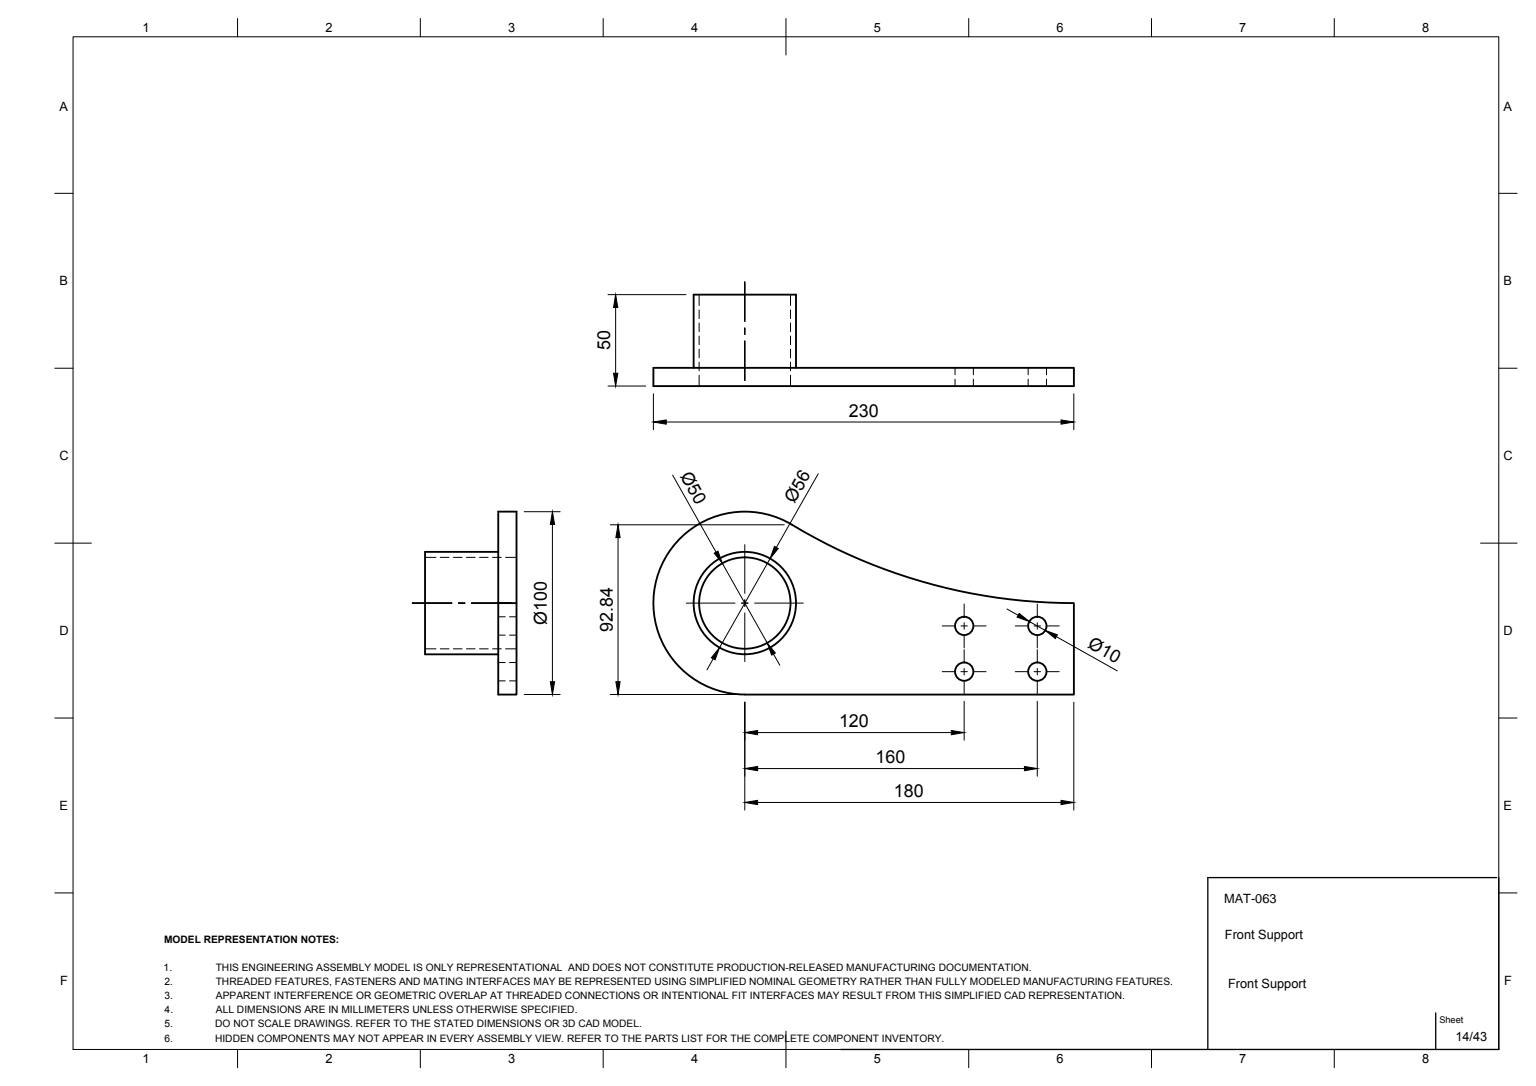
ISO-10303-21;
HEADER;
/* Generated by software containing ST-Developer
 * from STEP Tools, Inc. (www.steptools.com) 
 */

FILE_DESCRIPTION(
/* description */ (''),
/* implementation_level */ '2;1');

FILE_NAME(
/* name */ 'Front Support.step',
/* time_stamp */ '2026-10-24T09:43:01-07:00',
/* author */ (''),
/* organization */ (''),
/* preprocessor_version */ 'ST-DEVELOPER v20.2',
/* originating_system */ 'Autodesk Translation Framework v15.15.0.0',
/* authorisation */ '');

FILE_SCHEMA (('AUTOMOTIVE_DESIGN { 1 0 10303 214 3 1 1 }'));
ENDSEC;

DATA;
#10=MECHANICAL_DESIGN_GEOMETRIC_PRESENTATION_REPRESENTATION('',(#302),#11112);
#236=SHAPE_REPRESENTATION_RELATIONSHIP('SRR','None',#11262,#269);
#269=ADVANCED_BREP_SHAPE_REPRESENTATION('',(#335),#11107);
#302=STYLED_ITEM('',(#11426),#335);
#335=MANIFOLD_SOLID_BREP('Front Support',#6039);
#481=FACE_BOUND('',#1521,.T.);
#482=FACE_BOUND('',#1523,.T.);
#483=FACE_BOUND('',#1524,.T.);
#484=FACE_BOUND('',#1525,.T.);
#485=FACE_BOUND('',#1526,.T.);
#486=FACE_BOUND('',#1527,.T.);
#487=FACE_BOUND('',#1538,.T.);
#488=FACE_BOUND('',#1539,.T.);
#489=FACE_BOUND('',#1540,.T.);
#490=FACE_BOUND('',#1541,.T.);
#491=FACE_BOUND('',#1542,.T.);
#654=PLANE('',#7190);
#655=PLANE('',#7192);
#656=PLANE('',#7209);
#657=PLANE('',#7214);
#658=PLANE('',#7215);
#1013=FACE_OUTER_BOUND('',#1519,.T.);
#1014=FACE_OUTER_BOUND('',#1520,.T.);
#1015=FACE_OUTER_BOUND('',#1522,.T.);
#1016=FACE_OUTER_BOUND('',#1528,.T.);
#1017=FACE_OUTER_BOUND('',#1529,.T.);
#1018=FACE_OUTER_BOUND('',#1530,.T.);
#1019=FACE_OUTER_BOUND('',#1531,.T.);
#1020=FACE_OUTER_BOUND('',#1532,.T.);
#1021=FACE_OUTER_BOUND('',#1533,.T.);
#1022=FACE_OUTER_BOUND('',#1534,.T.);
#1023=FACE_OUTER_BOUND('',#1535,.T.);
#1024=FACE_OUTER_BOUND('',#1536,.T.);
#1025=FACE_OUTER_BOUND('',#1537,.T.);
#1519=EDGE_LOOP('',(#5409,#5410,#5411,#5412));
#1520=EDGE_LOOP('',(#5413));
#1521=EDGE_LOOP('',(#5414));
#1522=EDGE_LOOP('',(#5415,#5416,#5417,#5418));
#1523=EDGE_LOOP('',(#5419));
#1524=EDGE_LOOP('',(#5420));
#1525=EDGE_LOOP('',(#5421));
#1526=EDGE_LOOP('',(#5422));
#1527=EDGE_LOOP('',(#5423));
#1528=EDGE_LOOP('',(#5424,#5425,#5426,#5427));
#1529=EDGE_LOOP('',(#5428,#5429,#5430,#5431));
#1530=EDGE_LOOP('',(#5432,#5433,#5434,#5435));
#1531=EDGE_LOOP('',(#5436,#5437,#5438,#5439));
#1532=EDGE_LOOP('',(#5440,#5441,#5442,#5443));
#1533=EDGE_LOOP('',(#5444,#5445,#5446,#5447));
#1534=EDGE_LOOP('',(#5448,#5449,#5450,#5451));
#1535=EDGE_LOOP('',(#5452,#5453,#5454,#5455));
#1536=EDGE_LOOP('',(#5456,#5457,#5458,#5459));
#1537=EDGE_LOOP('',(#5460,#5461,#5462,#5463));
#1538=EDGE_LOOP('',(#5464));
#1539=EDGE_LOOP('',(#5465));
#1540=EDGE_LOOP('',(#5466));
#1541=EDGE_LOOP('',(#5467));
#1542=EDGE_LOOP('',(#5468));
#1898=LINE('',#10917,#2257);
#1899=LINE('',#10925,#2258);
#1900=LINE('',#10927,#2259);
#1901=LINE('',#10942,#2260);
#1902=LINE('',#10946,#2261);
#1903=LINE('',#10950,#2262);
#1904=LINE('',#10954,#2263);
#1905=LINE('',#10958,#2264);
#1906=LINE('',#10961,#2265);
#1907=LINE('',#10963,#2266);
#1908=LINE('',#10964,#2267);
#1909=LINE('',#10968,#2268);
#1910=LINE('',#10971,#2269);
#1911=LINE('',#10974,#2270);
#2257=VECTOR('',#9164,0.028);
#2258=VECTOR('',#9173,0.01);
#2259=VECTOR('',#9174,0.01);
#2260=VECTOR('',#9191,0.025);
#2261=VECTOR('',#9196,0.0049999999999998);
#2262=VECTOR('',#9201,0.005);
#2263=VECTOR('',#9206,0.0049999999999998);
#2264=VECTOR('',#9211,0.005);
#2265=VECTOR('',#9214,0.01);
#2266=VECTOR('',#9215,0.01);
#2267=VECTOR('',#9216,0.01);
#2268=VECTOR('',#9221,0.01);
#2269=VECTOR('',#9224,0.01);
#2270=VECTOR('',#9229,0.01);
#2656=CIRCLE('',#7188,0.028);
#2657=CIRCLE('',#7189,0.028);
#2658=CIRCLE('',#7191,0.025);
#2659=CIRCLE('',#7193,0.299);
#2660=CIRCLE('',#7194,0.05);
#2661=CIRCLE('',#7195,0.005);
#2662=CIRCLE('',#7196,0.0049999999999998);
#2663=CIRCLE('',#7197,0.005);
#2664=CIRCLE('',#7198,0.0049999999999998);
#2665=CIRCLE('',#7200,0.025);
#2666=CIRCLE('',#7202,0.0049999999999998);
#2667=CIRCLE('',#7204,0.005);
#2668=CIRCLE('',#7206,0.0049999999999998);
#2669=CIRCLE('',#7208,0.005);
#2670=CIRCLE('',#7211,0.299);
#2671=CIRCLE('',#7213,0.05);
#3150=VERTEX_POINT('',#10914);
#3151=VERTEX_POINT('',#10916);
#3152=VERTEX_POINT('',#10920);
#3153=VERTEX_POINT('',#10923);
#3154=VERTEX_POINT('',#10924);
#3155=VERTEX_POINT('',#10926);
#3156=VERTEX_POINT('',#10928);
#3157=VERTEX_POINT('',#10931);
#3158=VERTEX_POINT('',#10933);
#3159=VERTEX_POINT('',#10935);
#3160=VERTEX_POINT('',#10937);
#3161=VERTEX_POINT('',#10940);
#3162=VERTEX_POINT('',#10944);
#3163=VERTEX_POINT('',#10948);
#3164=VERTEX_POINT('',#10952);
#3165=VERTEX_POINT('',#10956);
#3166=VERTEX_POINT('',#10960);
#3167=VERTEX_POINT('',#10962);
#3168=VERTEX_POINT('',#10966);
#3169=VERTEX_POINT('',#10970);
#3908=EDGE_CURVE('',#3150,#3150,#2656,.F.);
#3909=EDGE_CURVE('',#3150,#3151,#1898,.T.);
#3910=EDGE_CURVE('',#3151,#3151,#2657,.T.);
#3911=EDGE_CURVE('',#3152,#3152,#2658,.F.);
#3912=EDGE_CURVE('',#3153,#3154,#1899,.T.);
#3913=EDGE_CURVE('',#3155,#3153,#1900,.T.);
#3914=EDGE_CURVE('',#3156,#3155,#2659,.T.);
#3915=EDGE_CURVE('',#3154,#3156,#2660,.F.);
#3916=EDGE_CURVE('',#3157,#3157,#2661,.T.);
#3917=EDGE_CURVE('',#3158,#3158,#2662,.T.);
#3918=EDGE_CURVE('',#3159,#3159,#2663,.T.);
#3919=EDGE_CURVE('',#3160,#3160,#2664,.T.);
#3920=EDGE_CURVE('',#3161,#3161,#2665,.T.);
#3921=EDGE_CURVE('',#3161,#3152,#1901,.T.);
#3922=EDGE_CURVE('',#3162,#3162,#2666,.T.);
#3923=EDGE_CURVE('',#3162,#3160,#1902,.T.);
#3924=EDGE_CURVE('',#3163,#3163,#2667,.T.);
#3925=EDGE_CURVE('',#3163,#3159,#1903,.T.);
#3926=EDGE_CURVE('',#3164,#3164,#2668,.T.);
#3927=EDGE_CURVE('',#3164,#3158,#1904,.T.);
#3928=EDGE_CURVE('',#3165,#3165,#2669,.T.);
#3929=EDGE_CURVE('',#3165,#3157,#1905,.T.);
#3930=EDGE_CURVE('',#3155,#3166,#1906,.T.);
#3931=EDGE_CURVE('',#3167,#3153,#1907,.T.);
#3932=EDGE_CURVE('',#3166,#3167,#1908,.T.);
#3933=EDGE_CURVE('',#3168,#3166,#2670,.T.);
#3934=EDGE_CURVE('',#3156,#3168,#1909,.F.);
#3935=EDGE_CURVE('',#3169,#3154,#1910,.F.);
#3936=EDGE_CURVE('',#3168,#3169,#2671,.T.);
#3937=EDGE_CURVE('',#3169,#3167,#1911,.T.);
#5409=ORIENTED_EDGE('',*,*,#3908,.T.);
#5410=ORIENTED_EDGE('',*,*,#3909,.T.);
#5411=ORIENTED_EDGE('',*,*,#3910,.T.);
#5412=ORIENTED_EDGE('',*,*,#3909,.F.);
#5413=ORIENTED_EDGE('',*,*,#3910,.F.);
#5414=ORIENTED_EDGE('',*,*,#3911,.T.);
#5415=ORIENTED_EDGE('',*,*,#3912,.F.);
#5416=ORIENTED_EDGE('',*,*,#3913,.F.);
#5417=ORIENTED_EDGE('',*,*,#3914,.F.);
#5418=ORIENTED_EDGE('',*,*,#3915,.F.);
#5419=ORIENTED_EDGE('',*,*,#3916,.F.);
#5420=ORIENTED_EDGE('',*,*,#3917,.F.);
#5421=ORIENTED_EDGE('',*,*,#3918,.F.);
#5422=ORIENTED_EDGE('',*,*,#3919,.F.);
#5423=ORIENTED_EDGE('',*,*,#3908,.F.);
#5424=ORIENTED_EDGE('',*,*,#3920,.F.);
#5425=ORIENTED_EDGE('',*,*,#3921,.T.);
#5426=ORIENTED_EDGE('',*,*,#3911,.F.);
#5427=ORIENTED_EDGE('',*,*,#3921,.F.);
#5428=ORIENTED_EDGE('',*,*,#3922,.F.);
#5429=ORIENTED_EDGE('',*,*,#3923,.T.);
#5430=ORIENTED_EDGE('',*,*,#3919,.T.);
#5431=ORIENTED_EDGE('',*,*,#3923,.F.);
#5432=ORIENTED_EDGE('',*,*,#3924,.F.);
#5433=ORIENTED_EDGE('',*,*,#3925,.T.);
#5434=ORIENTED_EDGE('',*,*,#3918,.T.);
#5435=ORIENTED_EDGE('',*,*,#3925,.F.);
#5436=ORIENTED_EDGE('',*,*,#3926,.F.);
#5437=ORIENTED_EDGE('',*,*,#3927,.T.);
#5438=ORIENTED_EDGE('',*,*,#3917,.T.);
#5439=ORIENTED_EDGE('',*,*,#3927,.F.);
#5440=ORIENTED_EDGE('',*,*,#3928,.F.);
#5441=ORIENTED_EDGE('',*,*,#3929,.T.);
#5442=ORIENTED_EDGE('',*,*,#3916,.T.);
#5443=ORIENTED_EDGE('',*,*,#3929,.F.);
#5444=ORIENTED_EDGE('',*,*,#3930,.F.);
#5445=ORIENTED_EDGE('',*,*,#3913,.T.);
#5446=ORIENTED_EDGE('',*,*,#3931,.F.);
#5447=ORIENTED_EDGE('',*,*,#3932,.F.);
#5448=ORIENTED_EDGE('',*,*,#3914,.T.);
#5449=ORIENTED_EDGE('',*,*,#3930,.T.);
#5450=ORIENTED_EDGE('',*,*,#3933,.F.);
#5451=ORIENTED_EDGE('',*,*,#3934,.F.);
#5452=ORIENTED_EDGE('',*,*,#3935,.T.);
#5453=ORIENTED_EDGE('',*,*,#3915,.T.);
#5454=ORIENTED_EDGE('',*,*,#3934,.T.);
#5455=ORIENTED_EDGE('',*,*,#3936,.T.);
#5456=ORIENTED_EDGE('',*,*,#3912,.T.);
#5457=ORIENTED_EDGE('',*,*,#3935,.F.);
#5458=ORIENTED_EDGE('',*,*,#3937,.T.);
#5459=ORIENTED_EDGE('',*,*,#3931,.T.);
#5460=ORIENTED_EDGE('',*,*,#3932,.T.);
#5461=ORIENTED_EDGE('',*,*,#3937,.F.);
#5462=ORIENTED_EDGE('',*,*,#3936,.F.);
#5463=ORIENTED_EDGE('',*,*,#3933,.T.);
#5464=ORIENTED_EDGE('',*,*,#3928,.T.);
#5465=ORIENTED_EDGE('',*,*,#3922,.T.);
#5466=ORIENTED_EDGE('',*,*,#3924,.T.);
#5467=ORIENTED_EDGE('',*,*,#3926,.T.);
#5468=ORIENTED_EDGE('',*,*,#3920,.T.);
#5633=CYLINDRICAL_SURFACE('',#7187,0.028);
#5634=CYLINDRICAL_SURFACE('',#7199,0.025);
#5635=CYLINDRICAL_SURFACE('',#7201,0.0049999999999998);
#5636=CYLINDRICAL_SURFACE('',#7203,0.005);
#5637=CYLINDRICAL_SURFACE('',#7205,0.0049999999999998);
#5638=CYLINDRICAL_SURFACE('',#7207,0.005);
#5639=CYLINDRICAL_SURFACE('',#7210,0.299);
#5640=CYLINDRICAL_SURFACE('',#7212,0.05);
#5986=ADVANCED_FACE('',(#1013),#5633,.T.);
#5987=ADVANCED_FACE('',(#1014,#481),#654,.T.);
#5988=ADVANCED_FACE('',(#1015,#482,#483,#484,#485,#486),#655,.F.);
#5989=ADVANCED_FACE('',(#1016),#5634,.F.);
#5990=ADVANCED_FACE('',(#1017),#5635,.F.);
#5991=ADVANCED_FACE('',(#1018),#5636,.F.);
#5992=ADVANCED_FACE('',(#1019),#5637,.F.);
#5993=ADVANCED_FACE('',(#1020),#5638,.F.);
#5994=ADVANCED_FACE('',(#1021),#656,.F.);
#5995=ADVANCED_FACE('',(#1022),#5639,.F.);
#5996=ADVANCED_FACE('',(#1023),#5640,.T.);
#5997=ADVANCED_FACE('',(#1024),#657,.T.);
#5998=ADVANCED_FACE('',(#1025,#487,#488,#489,#490,#491),#658,.T.);
#6039=CLOSED_SHELL('',(#5986,#5987,#5988,#5989,#5990,#5991,#5992,#5993,
#5994,#5995,#5996,#5997,#5998));
#7186=AXIS2_PLACEMENT_3D('',#10912,#9158,#9159);
#7187=AXIS2_PLACEMENT_3D('',#10913,#9160,#9161);
#7188=AXIS2_PLACEMENT_3D('',#10915,#9162,#9163);
#7189=AXIS2_PLACEMENT_3D('',#10918,#9165,#9166);
#7190=AXIS2_PLACEMENT_3D('',#10919,#9167,#9168);
#7191=AXIS2_PLACEMENT_3D('',#10921,#9169,#9170);
#7192=AXIS2_PLACEMENT_3D('',#10922,#9171,#9172);
#7193=AXIS2_PLACEMENT_3D('',#10929,#9175,#9176);
#7194=AXIS2_PLACEMENT_3D('',#10930,#9177,#9178);
#7195=AXIS2_PLACEMENT_3D('',#10932,#9179,#9180);
#7196=AXIS2_PLACEMENT_3D('',#10934,#9181,#9182);
#7197=AXIS2_PLACEMENT_3D('',#10936,#9183,#9184);
#7198=AXIS2_PLACEMENT_3D('',#10938,#9185,#9186);
#7199=AXIS2_PLACEMENT_3D('',#10939,#9187,#9188);
#7200=AXIS2_PLACEMENT_3D('',#10941,#9189,#9190);
#7201=AXIS2_PLACEMENT_3D('',#10943,#9192,#9193);
#7202=AXIS2_PLACEMENT_3D('',#10945,#9194,#9195);
#7203=AXIS2_PLACEMENT_3D('',#10947,#9197,#9198);
#7204=AXIS2_PLACEMENT_3D('',#10949,#9199,#9200);
#7205=AXIS2_PLACEMENT_3D('',#10951,#9202,#9203);
#7206=AXIS2_PLACEMENT_3D('',#10953,#9204,#9205);
#7207=AXIS2_PLACEMENT_3D('',#10955,#9207,#9208);
#7208=AXIS2_PLACEMENT_3D('',#10957,#9209,#9210);
#7209=AXIS2_PLACEMENT_3D('',#10959,#9212,#9213);
#7210=AXIS2_PLACEMENT_3D('',#10965,#9217,#9218);
#7211=AXIS2_PLACEMENT_3D('',#10967,#9219,#9220);
#7212=AXIS2_PLACEMENT_3D('',#10969,#9222,#9223);
#7213=AXIS2_PLACEMENT_3D('',#10972,#9225,#9226);
#7214=AXIS2_PLACEMENT_3D('',#10973,#9227,#9228);
#7215=AXIS2_PLACEMENT_3D('',#10975,#9230,#9231);
#9158=DIRECTION('axis',(0.,0.,1.));
#9159=DIRECTION('refdir',(1.,0.,0.));
#9160=DIRECTION('center_axis',(-1.,0.,0.));
#9161=DIRECTION('ref_axis',(0.,0.,1.));
#9162=DIRECTION('center_axis',(-1.,0.,0.));
#9163=DIRECTION('ref_axis',(0.,0.,1.));
#9164=DIRECTION('',(1.,0.,0.));
#9165=DIRECTION('center_axis',(-1.,0.,0.));
#9166=DIRECTION('ref_axis',(0.,0.,1.));
#9167=DIRECTION('center_axis',(1.,-9.9268665898833E-16,1.01959257413342E-15));
#9168=DIRECTION('ref_axis',(1.01959257413342E-15,0.,-1.));
#9169=DIRECTION('center_axis',(1.,0.,0.));
#9170=DIRECTION('ref_axis',(0.,0.,-1.));
#9171=DIRECTION('center_axis',(-1.,0.,0.));
#9172=DIRECTION('ref_axis',(0.,0.,1.));
#9173=DIRECTION('',(0.,0.,1.));
#9174=DIRECTION('',(0.,-1.,1.98951966438983E-14));
#9175=DIRECTION('center_axis',(1.,0.,0.));
#9176=DIRECTION('ref_axis',(0.,0.,-1.));
#9177=DIRECTION('center_axis',(1.,0.,0.));
#9178=DIRECTION('ref_axis',(0.,0.,-1.));
#9179=DIRECTION('center_axis',(1.,0.,0.));
#9180=DIRECTION('ref_axis',(0.,0.,-1.));
#9181=DIRECTION('center_axis',(1.,0.,0.));
#9182=DIRECTION('ref_axis',(0.,0.,-1.));
#9183=DIRECTION('center_axis',(1.,0.,0.));
#9184=DIRECTION('ref_axis',(0.,0.,-1.));
#9185=DIRECTION('center_axis',(1.,0.,0.));
#9186=DIRECTION('ref_axis',(0.,0.,-1.));
#9187=DIRECTION('center_axis',(1.,0.,0.));
#9188=DIRECTION('ref_axis',(0.,0.,-1.));
#9189=DIRECTION('center_axis',(1.,0.,0.));
#9190=DIRECTION('ref_axis',(0.,0.,-1.));
#9191=DIRECTION('',(1.,0.,0.));
#9192=DIRECTION('center_axis',(1.,0.,0.));
#9193=DIRECTION('ref_axis',(0.,0.,-1.));
#9194=DIRECTION('center_axis',(1.,0.,0.));
#9195=DIRECTION('ref_axis',(0.,0.,-1.));
#9196=DIRECTION('',(1.,0.,0.));
#9197=DIRECTION('center_axis',(1.,0.,0.));
#9198=DIRECTION('ref_axis',(0.,0.,-1.));
#9199=DIRECTION('center_axis',(1.,0.,0.));
#9200=DIRECTION('ref_axis',(0.,0.,-1.));
#9201=DIRECTION('',(1.,0.,0.));
#9202=DIRECTION('center_axis',(1.,0.,0.));
#9203=DIRECTION('ref_axis',(0.,0.,-1.));
#9204=DIRECTION('center_axis',(1.,0.,0.));
#9205=DIRECTION('ref_axis',(0.,0.,-1.));
#9206=DIRECTION('',(1.,0.,0.));
#9207=DIRECTION('center_axis',(1.,0.,0.));
#9208=DIRECTION('ref_axis',(0.,0.,-1.));
#9209=DIRECTION('center_axis',(1.,0.,0.));
#9210=DIRECTION('ref_axis',(0.,0.,-1.));
#9211=DIRECTION('',(1.,0.,0.));
#9212=DIRECTION('center_axis',(2.20458572024499E-15,5.64627709665039E-16,
1.));
#9213=DIRECTION('ref_axis',(1.,5.1073991127734E-47,-2.20458572024499E-15));
#9214=DIRECTION('',(-1.,0.,0.));
#9215=DIRECTION('',(1.,0.,0.));
#9216=DIRECTION('',(0.,-1.,0.));
#9217=DIRECTION('center_axis',(1.,0.,0.));
#9218=DIRECTION('ref_axis',(0.,0.,-1.));
#9219=DIRECTION('center_axis',(1.,0.,0.));
#9220=DIRECTION('ref_axis',(0.,0.,-1.));
#9221=DIRECTION('',(1.,0.,0.));
#9222=DIRECTION('center_axis',(1.,0.,0.));
#9223=DIRECTION('ref_axis',(0.,0.267643864798619,0.963517909348684));
#9224=DIRECTION('',(-1.,0.,0.));
#9225=DIRECTION('center_axis',(1.,0.,0.));
#9226=DIRECTION('ref_axis',(0.,0.,-1.));
#9227=DIRECTION('center_axis',(3.68752646949032E-16,-1.,-1.69617406532146E-17));
#9228=DIRECTION('ref_axis',(1.,3.68752646949032E-16,0.));
#9229=DIRECTION('',(0.,0.,-1.));
#9230=DIRECTION('center_axis',(-1.,0.,0.));
#9231=DIRECTION('ref_axis',(0.,0.,1.));
#10912=CARTESIAN_POINT('',(0.,0.,0.));
#10913=CARTESIAN_POINT('Origin',(-0.46,0.35,1.1));
#10914=CARTESIAN_POINT('',(-0.5,0.35,1.072));
#10915=CARTESIAN_POINT('Origin',(-0.5,0.35,1.1));
#10916=CARTESIAN_POINT('',(-0.46,0.35,1.072));
#10917=CARTESIAN_POINT('',(-0.46,0.35,1.072));
#10918=CARTESIAN_POINT('Origin',(-0.46,0.35,1.1));
#10919=CARTESIAN_POINT('Origin',(-0.46,0.35,1.1));
#10920=CARTESIAN_POINT('',(-0.46,0.35,1.125));
#10921=CARTESIAN_POINT('Origin',(-0.46,0.35,1.1));
#10922=CARTESIAN_POINT('Origin',(-0.5,0.35003431001795,1.0350379192153));
#10923=CARTESIAN_POINT('',(-0.5,0.3,0.92));
#10924=CARTESIAN_POINT('',(-0.500000000000071,0.3,1.10000000002108));
#10925=CARTESIAN_POINT('',(-0.5,0.3,0.92));
#10926=CARTESIAN_POINT('',(-0.5,0.349999999999381,0.92));
#10927=CARTESIAN_POINT('',(-0.5,0.3499999998929,0.919999999999999));
#10928=CARTESIAN_POINT('',(-0.5,0.392836676173592,1.07421203431058));
#10929=CARTESIAN_POINT('Origin',(-0.5,0.649,0.92));
#10930=CARTESIAN_POINT('Origin',(-0.5,0.35,1.1));
#10931=CARTESIAN_POINT('',(-0.5,0.3125,0.985));
#10932=CARTESIAN_POINT('Origin',(-0.5,0.3125,0.98));
#10933=CARTESIAN_POINT('',(-0.5,0.3375,0.945));
#10934=CARTESIAN_POINT('Origin',(-0.5,0.3375,0.94));
#10935=CARTESIAN_POINT('',(-0.5,0.3375,0.985));
#10936=CARTESIAN_POINT('Origin',(-0.5,0.3375,0.98));
#10937=CARTESIAN_POINT('',(-0.5,0.3125,0.945));
#10938=CARTESIAN_POINT('Origin',(-0.5,0.3125,0.94));
#10939=CARTESIAN_POINT('Origin',(-0.51,0.35,1.1));
#10940=CARTESIAN_POINT('',(-0.51,0.35,1.125));
#10941=CARTESIAN_POINT('Origin',(-0.51,0.35,1.1));
#10942=CARTESIAN_POINT('',(-0.51,0.35,1.125));
#10943=CARTESIAN_POINT('Origin',(-0.51,0.3125,0.94));
#10944=CARTESIAN_POINT('',(-0.51,0.3125,0.945));
#10945=CARTESIAN_POINT('Origin',(-0.51,0.3125,0.94));
#10946=CARTESIAN_POINT('',(-0.51,0.3125,0.945));
#10947=CARTESIAN_POINT('Origin',(-0.51,0.3375,0.98));
#10948=CARTESIAN_POINT('',(-0.51,0.3375,0.985));
#10949=CARTESIAN_POINT('Origin',(-0.51,0.3375,0.98));
#10950=CARTESIAN_POINT('',(-0.51,0.3375,0.985));
#10951=CARTESIAN_POINT('Origin',(-0.51,0.3375,0.94));
#10952=CARTESIAN_POINT('',(-0.51,0.3375,0.945));
#10953=CARTESIAN_POINT('Origin',(-0.51,0.3375,0.94));
#10954=CARTESIAN_POINT('',(-0.51,0.3375,0.945));
#10955=CARTESIAN_POINT('Origin',(-0.51,0.3125,0.98));
#10956=CARTESIAN_POINT('',(-0.51,0.3125,0.985));
#10957=CARTESIAN_POINT('Origin',(-0.51,0.3125,0.98));
#10958=CARTESIAN_POINT('',(-0.51,0.3125,0.985));
#10959=CARTESIAN_POINT('Origin',(-0.505,0.325,0.92));
#10960=CARTESIAN_POINT('',(-0.51,0.349999999999358,0.92));
#10961=CARTESIAN_POINT('',(-0.500000000000001,0.35,0.92));
#10962=CARTESIAN_POINT('',(-0.51,0.3,0.92));
#10963=CARTESIAN_POINT('',(-0.510000000000001,0.3,0.92));
#10964=CARTESIAN_POINT('',(-0.510000000000001,0.34999999975,0.92));
#10965=CARTESIAN_POINT('Origin',(-0.51,0.649,0.92));
#10966=CARTESIAN_POINT('',(-0.51,0.392836676173675,1.07421203431072));
#10967=CARTESIAN_POINT('Origin',(-0.51,0.649,0.92));
#10968=CARTESIAN_POINT('',(-0.50999999975,0.392836676172712,1.07421203430912));
#10969=CARTESIAN_POINT('Origin',(-0.51,0.35,1.1));
#10970=CARTESIAN_POINT('',(-0.510000000000001,0.3,1.10000000001774));
#10971=CARTESIAN_POINT('',(-0.50000000025,0.3,1.10000000001923));
#10972=CARTESIAN_POINT('Origin',(-0.51,0.35,1.1));
#10973=CARTESIAN_POINT('Origin',(-0.505,0.3,1.01));
#10974=CARTESIAN_POINT('',(-0.510000000000002,0.3,1.1));
#10975=CARTESIAN_POINT('Origin',(-0.51,0.35003431001795,1.0350379192153));
#11068=UNCERTAINTY_MEASURE_WITH_UNIT(LENGTH_MEASURE(1.E-5),#11113,
'DISTANCE_ACCURACY_VALUE',
'Maximum model space distance between geometric entities at asserted c
onnectivities');
#11073=UNCERTAINTY_MEASURE_WITH_UNIT(LENGTH_MEASURE(1.E-5),#11113,
'DISTANCE_ACCURACY_VALUE',
'Maximum model space distance between geometric entities at asserted c
onnectivities');
#11107=(
GEOMETRIC_REPRESENTATION_CONTEXT(3)
GLOBAL_UNCERTAINTY_ASSIGNED_CONTEXT((#11068))
GLOBAL_UNIT_ASSIGNED_CONTEXT((#11113,#11114,#11115))
REPRESENTATION_CONTEXT('','3D')
);
#11112=(
GEOMETRIC_REPRESENTATION_CONTEXT(3)
GLOBAL_UNCERTAINTY_ASSIGNED_CONTEXT((#11073))
GLOBAL_UNIT_ASSIGNED_CONTEXT((#11113,#11114,#11115))
REPRESENTATION_CONTEXT('','3D')
);
#11113=(
LENGTH_UNIT()
NAMED_UNIT(*)
SI_UNIT($,.METRE.)
);
#11114=(
NAMED_UNIT(*)
PLANE_ANGLE_UNIT()
SI_UNIT($,.RADIAN.)
);
#11115=(
NAMED_UNIT(*)
SI_UNIT($,.STERADIAN.)
SOLID_ANGLE_UNIT()
);
#11149=SHAPE_DEFINITION_REPRESENTATION(#11205,#11262);
#11205=PRODUCT_DEFINITION_SHAPE('',$,#11301);
#11262=SHAPE_REPRESENTATION('',(#7186),#11107);
#11267=PRODUCT_DEFINITION_CONTEXT('part definition',#11383,'design');
#11301=PRODUCT_DEFINITION('Front Support','Front Support',#11339,#11267);
#11339=PRODUCT_DEFINITION_FORMATION('',$,#11418);
#11383=APPLICATION_CONTEXT(
'Core Data for Automotive Mechanical Design Process');
#11384=PRODUCT_CONTEXT('part definition',#11383,'mechanical');
#11418=PRODUCT('Front Support','Front Support',
'front_sup__ DE     7651',(#11384));
#11426=PRESENTATION_STYLE_ASSIGNMENT((#11430));
#11430=SURFACE_STYLE_USAGE(.BOTH.,#11434);
#11434=SURFACE_SIDE_STYLE('',(#11438));
#11438=SURFACE_STYLE_FILL_AREA(#11442);
#11442=FILL_AREA_STYLE('Opaque(202,209,238)',(#11446));
#11446=FILL_AREA_STYLE_COLOUR('Opaque(202,209,238)',#11450);
#11450=COLOUR_RGB('Opaque(202,209,238)',0.792156862745098,0.819607843137255,
0.933333333333333);
ENDSEC;
END-ISO-10303-21;
